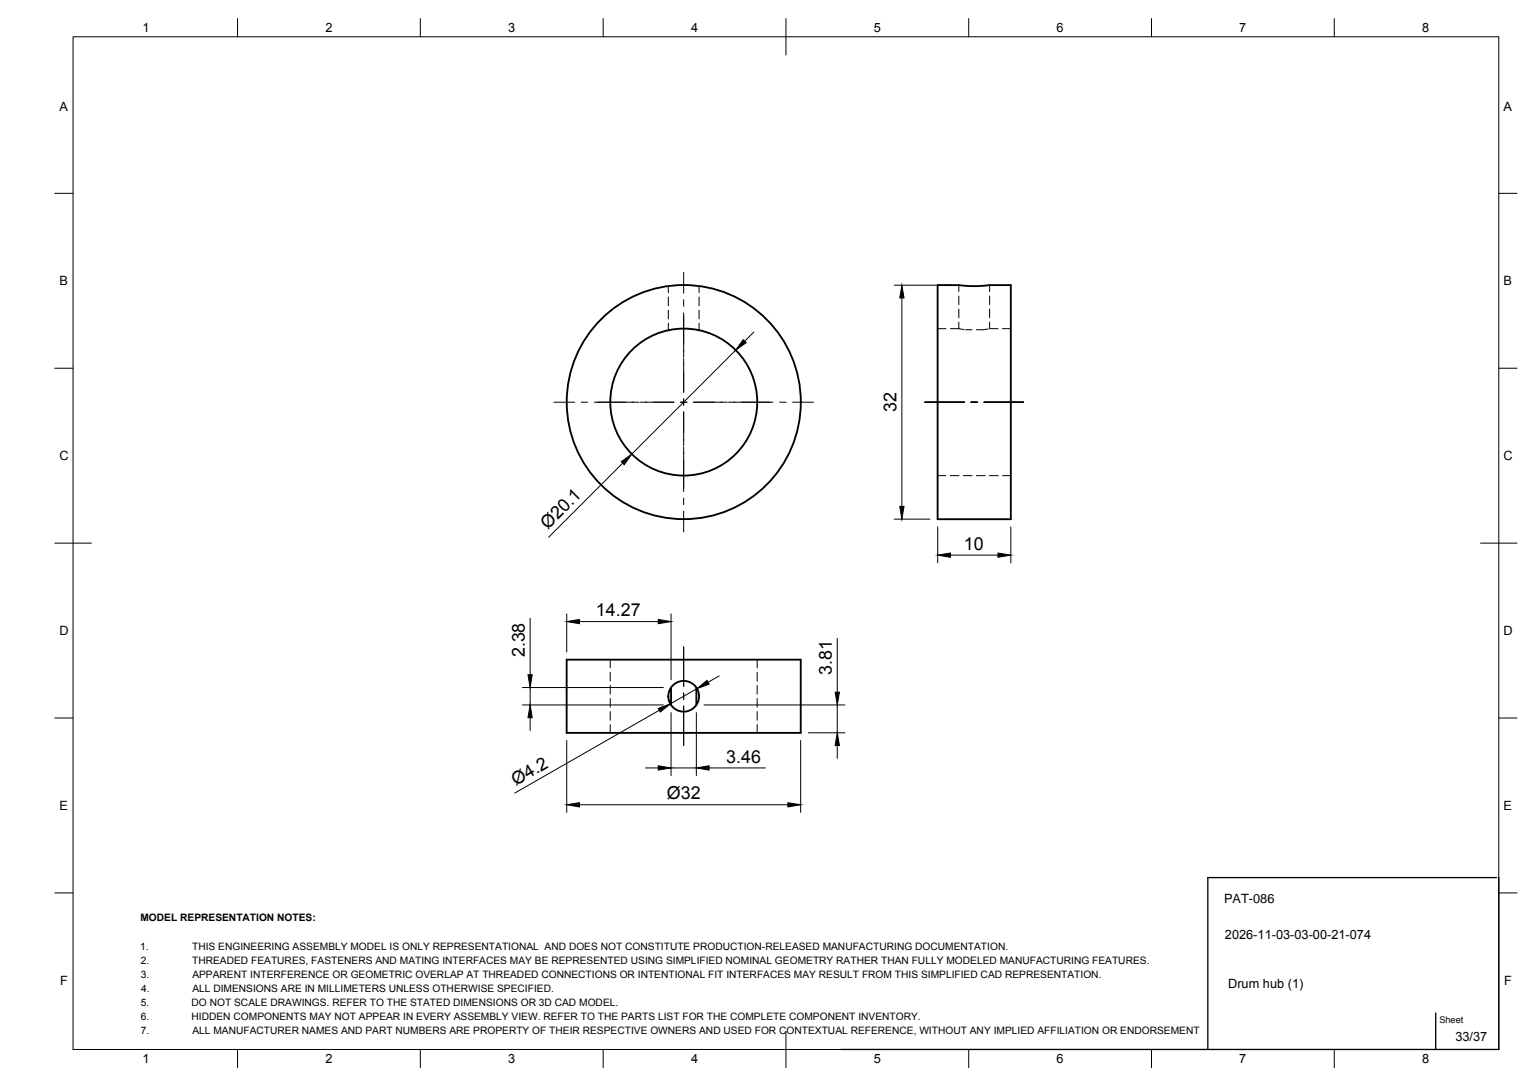
ISO-10303-21;
HEADER;
/* Generated by software containing ST-Developer
 * from STEP Tools, Inc. (www.steptools.com) 
 */

FILE_DESCRIPTION(
/* description */ ('Ratchet and pawl hand winch drum'),
/* implementation_level */ '2;1');

FILE_NAME(
/* name */ 'Drum hub (1).step',
/* time_stamp */ '2026-10-27T12:42:58-07:00',
/* author */ (''),
/* organization */ (''),
/* preprocessor_version */ 'ST-DEVELOPER v20.2',
/* originating_system */ 'Autodesk Translation Framework v15.17.0.0',
/* authorisation */ '');

FILE_SCHEMA (('AUTOMOTIVE_DESIGN { 1 0 10303 214 3 1 1 }'));
ENDSEC;

DATA;
#10=MECHANICAL_DESIGN_GEOMETRIC_PRESENTATION_REPRESENTATION('',(#417),#11801);
#309=B_SPLINE_CURVE_WITH_KNOTS('',3,(#10928,#10929,#10930,#10931,#10932,
#10933,#10934,#10935,#10936,#10937,#10938,#10939,#10940,#10941),
 .UNSPECIFIED.,.F.,.F.,(4,2,2,2,2,2,4),(0.756005737987023,0.793568827564648,
0.872922520054203,0.952276212543758,1.03162990503331,1.11098359752287,1.1485466871005),
 .UNSPECIFIED.);
#310=B_SPLINE_CURVE_WITH_KNOTS('',3,(#10947,#10948,#10949,#10950,#10951,
#10952,#10953,#10954,#10955,#10956,#10957,#10958,#10959,#10960,#10961,#10962,
#10963,#10964),.UNSPECIFIED.,.F.,.F.,(4,2,2,2,2,2,2,2,4),(0.,0.0792028026112442,
0.158405605222488,0.237607602356378,0.316809599490267,0.396011596624156,
0.475213593758046,0.55441639636929,0.633619198980534),.UNSPECIFIED.);
#311=B_SPLINE_CURVE_WITH_KNOTS('',3,(#10965,#10966,#10967,#10968,#10969,
#10970,#10971,#10972,#10973,#10974,#10975,#10976,#10977,#10978,#10979,#10980,
#10981,#10982),.UNSPECIFIED.,.F.,.F.,(4,2,2,2,2,2,2,2,4),(0.633619198980534,
0.712822001591778,0.792024804203022,0.871226801336912,0.950428798470801,
1.02963079560469,1.10883279273858,1.18803559534982,1.26723839796107),
 .UNSPECIFIED.);
#312=B_SPLINE_CURVE_WITH_KNOTS('',3,(#10985,#10986,#10987,#10988,#10989,
#10990,#10991,#10992,#10993,#10994,#10995,#10996,#10997,#10998),
 .UNSPECIFIED.,.F.,.F.,(4,2,2,2,2,2,4),(0.121154929624518,0.158718019202143,
0.238071711691698,0.317425404181253,0.396779096670807,0.476132789160362,
0.513695878737989),.UNSPECIFIED.);
#348=SHAPE_REPRESENTATION_RELATIONSHIP('SRR','None',#11976,#382);
#382=ADVANCED_BREP_SHAPE_REPRESENTATION('',(#450),#11793);
#417=STYLED_ITEM('',(#12199),#450);
#450=MANIFOLD_SOLID_BREP('Body1',#6296);
#582=FACE_BOUND('',#1565,.T.);
#583=FACE_BOUND('',#1567,.T.);
#584=FACE_BOUND('',#1569,.T.);
#585=FACE_BOUND('',#1571,.T.);
#746=PLANE('',#7129);
#747=PLANE('',#7134);
#748=PLANE('',#7141);
#749=PLANE('',#7142);
#1079=FACE_OUTER_BOUND('',#1561,.T.);
#1080=FACE_OUTER_BOUND('',#1562,.T.);
#1081=FACE_OUTER_BOUND('',#1563,.T.);
#1082=FACE_OUTER_BOUND('',#1564,.T.);
#1083=FACE_OUTER_BOUND('',#1566,.T.);
#1084=FACE_OUTER_BOUND('',#1568,.T.);
#1085=FACE_OUTER_BOUND('',#1570,.T.);
#1561=EDGE_LOOP('',(#5239,#5240));
#1562=EDGE_LOOP('',(#5241,#5242,#5243,#5244,#5245,#5246,#5247,#5248,#5249));
#1563=EDGE_LOOP('',(#5250,#5251,#5252));
#1564=EDGE_LOOP('',(#5253,#5254,#5255,#5256));
#1565=EDGE_LOOP('',(#5257,#5258,#5259,#5260));
#1566=EDGE_LOOP('',(#5261,#5262,#5263,#5264));
#1567=EDGE_LOOP('',(#5265,#5266));
#1568=EDGE_LOOP('',(#5267));
#1569=EDGE_LOOP('',(#5268));
#1570=EDGE_LOOP('',(#5269));
#1571=EDGE_LOOP('',(#5270));
#1980=LINE('',#10924,#2491);
#1981=LINE('',#10945,#2492);
#1982=LINE('',#11000,#2493);
#1983=LINE('',#11005,#2494);
#1984=LINE('',#11011,#2495);
#2491=VECTOR('',#8543,1.);
#2492=VECTOR('',#8550,0.21);
#2493=VECTOR('',#8555,1.);
#2494=VECTOR('',#8560,1.005);
#2495=VECTOR('',#8567,1.6);
#2896=CIRCLE('',#7130,0.21);
#2897=CIRCLE('',#7132,0.21);
#2898=CIRCLE('',#7133,0.21);
#2899=CIRCLE('',#7136,1.005);
#2900=CIRCLE('',#7137,1.005);
#2901=CIRCLE('',#7139,1.6);
#2902=CIRCLE('',#7140,1.6);
#3279=VERTEX_POINT('',#10922);
#3280=VERTEX_POINT('',#10923);
#3281=VERTEX_POINT('',#10927);
#3282=VERTEX_POINT('',#10942);
#3283=VERTEX_POINT('',#10944);
#3284=VERTEX_POINT('',#10946);
#3285=VERTEX_POINT('',#10983);
#3286=VERTEX_POINT('',#11002);
#3287=VERTEX_POINT('',#11004);
#3288=VERTEX_POINT('',#11008);
#3289=VERTEX_POINT('',#11010);
#3963=EDGE_CURVE('',#3279,#3280,#1980,.T.);
#3964=EDGE_CURVE('',#3279,#3280,#2896,.T.);
#3965=EDGE_CURVE('',#3281,#3279,#309,.T.);
#3966=EDGE_CURVE('',#3282,#3281,#2897,.T.);
#3967=EDGE_CURVE('',#3282,#3283,#1981,.T.);
#3968=EDGE_CURVE('',#3284,#3283,#310,.T.);
#3969=EDGE_CURVE('',#3283,#3284,#311,.T.);
#3970=EDGE_CURVE('',#3285,#3282,#2898,.T.);
#3971=EDGE_CURVE('',#3280,#3285,#312,.T.);
#3972=EDGE_CURVE('',#3285,#3281,#1982,.T.);
#3973=EDGE_CURVE('',#3286,#3286,#2899,.T.);
#3974=EDGE_CURVE('',#3286,#3287,#1983,.T.);
#3975=EDGE_CURVE('',#3287,#3287,#2900,.T.);
#3976=EDGE_CURVE('',#3288,#3288,#2901,.T.);
#3977=EDGE_CURVE('',#3288,#3289,#1984,.T.);
#3978=EDGE_CURVE('',#3289,#3289,#2902,.T.);
#5239=ORIENTED_EDGE('',*,*,#3963,.F.);
#5240=ORIENTED_EDGE('',*,*,#3964,.T.);
#5241=ORIENTED_EDGE('',*,*,#3965,.F.);
#5242=ORIENTED_EDGE('',*,*,#3966,.F.);
#5243=ORIENTED_EDGE('',*,*,#3967,.T.);
#5244=ORIENTED_EDGE('',*,*,#3968,.F.);
#5245=ORIENTED_EDGE('',*,*,#3969,.F.);
#5246=ORIENTED_EDGE('',*,*,#3967,.F.);
#5247=ORIENTED_EDGE('',*,*,#3970,.F.);
#5248=ORIENTED_EDGE('',*,*,#3971,.F.);
#5249=ORIENTED_EDGE('',*,*,#3964,.F.);
#5250=ORIENTED_EDGE('',*,*,#3972,.F.);
#5251=ORIENTED_EDGE('',*,*,#3970,.T.);
#5252=ORIENTED_EDGE('',*,*,#3966,.T.);
#5253=ORIENTED_EDGE('',*,*,#3973,.F.);
#5254=ORIENTED_EDGE('',*,*,#3974,.T.);
#5255=ORIENTED_EDGE('',*,*,#3975,.T.);
#5256=ORIENTED_EDGE('',*,*,#3974,.F.);
#5257=ORIENTED_EDGE('',*,*,#3971,.T.);
#5258=ORIENTED_EDGE('',*,*,#3972,.T.);
#5259=ORIENTED_EDGE('',*,*,#3965,.T.);
#5260=ORIENTED_EDGE('',*,*,#3963,.T.);
#5261=ORIENTED_EDGE('',*,*,#3976,.F.);
#5262=ORIENTED_EDGE('',*,*,#3977,.T.);
#5263=ORIENTED_EDGE('',*,*,#3978,.T.);
#5264=ORIENTED_EDGE('',*,*,#3977,.F.);
#5265=ORIENTED_EDGE('',*,*,#3968,.T.);
#5266=ORIENTED_EDGE('',*,*,#3969,.T.);
#5267=ORIENTED_EDGE('',*,*,#3976,.T.);
#5268=ORIENTED_EDGE('',*,*,#3973,.T.);
#5269=ORIENTED_EDGE('',*,*,#3978,.F.);
#5270=ORIENTED_EDGE('',*,*,#3975,.F.);
#5893=CYLINDRICAL_SURFACE('',#7131,0.21);
#5894=CYLINDRICAL_SURFACE('',#7135,1.005);
#5895=CYLINDRICAL_SURFACE('',#7138,1.6);
#6149=ADVANCED_FACE('',(#1079),#746,.T.);
#6150=ADVANCED_FACE('',(#1080),#5893,.F.);
#6151=ADVANCED_FACE('',(#1081),#747,.T.);
#6152=ADVANCED_FACE('',(#1082,#582),#5894,.F.);
#6153=ADVANCED_FACE('',(#1083,#583),#5895,.T.);
#6154=ADVANCED_FACE('',(#1084,#584),#748,.T.);
#6155=ADVANCED_FACE('',(#1085,#585),#749,.F.);
#6296=CLOSED_SHELL('',(#6149,#6150,#6151,#6152,#6153,#6154,#6155));
#7128=AXIS2_PLACEMENT_3D('',#10920,#8539,#8540);
#7129=AXIS2_PLACEMENT_3D('',#10921,#8541,#8542);
#7130=AXIS2_PLACEMENT_3D('',#10925,#8544,#8545);
#7131=AXIS2_PLACEMENT_3D('',#10926,#8546,#8547);
#7132=AXIS2_PLACEMENT_3D('',#10943,#8548,#8549);
#7133=AXIS2_PLACEMENT_3D('',#10984,#8551,#8552);
#7134=AXIS2_PLACEMENT_3D('',#10999,#8553,#8554);
#7135=AXIS2_PLACEMENT_3D('',#11001,#8556,#8557);
#7136=AXIS2_PLACEMENT_3D('',#11003,#8558,#8559);
#7137=AXIS2_PLACEMENT_3D('',#11006,#8561,#8562);
#7138=AXIS2_PLACEMENT_3D('',#11007,#8563,#8564);
#7139=AXIS2_PLACEMENT_3D('',#11009,#8565,#8566);
#7140=AXIS2_PLACEMENT_3D('',#11012,#8568,#8569);
#7141=AXIS2_PLACEMENT_3D('',#11013,#8570,#8571);
#7142=AXIS2_PLACEMENT_3D('',#11014,#8572,#8573);
#8539=DIRECTION('axis',(0.,0.,1.));
#8540=DIRECTION('refdir',(1.,0.,0.));
#8541=DIRECTION('center_axis',(0.,0.,1.));
#8542=DIRECTION('ref_axis',(1.,0.,0.));
#8543=DIRECTION('',(0.,1.,0.));
#8544=DIRECTION('center_axis',(0.,0.,1.));
#8545=DIRECTION('ref_axis',(1.,0.,0.));
#8546=DIRECTION('center_axis',(0.,0.,1.));
#8547=DIRECTION('ref_axis',(1.,0.,0.));
#8548=DIRECTION('center_axis',(0.,0.,1.));
#8549=DIRECTION('ref_axis',(1.,0.,0.));
#8550=DIRECTION('',(0.,0.,1.));
#8551=DIRECTION('center_axis',(0.,0.,1.));
#8552=DIRECTION('ref_axis',(1.,0.,0.));
#8553=DIRECTION('center_axis',(0.,0.,1.));
#8554=DIRECTION('ref_axis',(1.,0.,0.));
#8555=DIRECTION('',(0.,-1.,0.));
#8556=DIRECTION('center_axis',(0.,1.,0.));
#8557=DIRECTION('ref_axis',(1.,0.,0.));
#8558=DIRECTION('center_axis',(0.,-1.,0.));
#8559=DIRECTION('ref_axis',(1.,0.,0.));
#8560=DIRECTION('',(0.,-1.,0.));
#8561=DIRECTION('center_axis',(0.,-1.,0.));
#8562=DIRECTION('ref_axis',(1.,0.,0.));
#8563=DIRECTION('center_axis',(0.,1.,0.));
#8564=DIRECTION('ref_axis',(1.,0.,0.));
#8565=DIRECTION('center_axis',(0.,1.,0.));
#8566=DIRECTION('ref_axis',(1.,0.,0.));
#8567=DIRECTION('',(0.,-1.,0.));
#8568=DIRECTION('center_axis',(0.,1.,0.));
#8569=DIRECTION('ref_axis',(1.,0.,0.));
#8570=DIRECTION('center_axis',(0.,1.,0.));
#8571=DIRECTION('ref_axis',(1.,0.,0.));
#8572=DIRECTION('center_axis',(0.,1.,0.));
#8573=DIRECTION('ref_axis',(1.,0.,0.));
#10920=CARTESIAN_POINT('',(0.,0.,0.));
#10921=CARTESIAN_POINT('Origin',(0.,12.5,7.52));
#10922=CARTESIAN_POINT('',(0.172988438920056,12.3809411910021,7.52));
#10923=CARTESIAN_POINT('',(0.172988438920056,12.6190588089979,7.52));
#10924=CARTESIAN_POINT('',(0.172988438920056,12.,7.52));
#10925=CARTESIAN_POINT('Origin',(0.,12.5,7.52));
#10926=CARTESIAN_POINT('Origin',(0.,12.5,7.52));
#10927=CARTESIAN_POINT('',(-0.172988438920056,12.3809411910021,7.52));
#10928=CARTESIAN_POINT('Ctrl Pts',(-0.172988438920057,12.3809411910021,
7.52));
#10929=CARTESIAN_POINT('Ctrl Pts',(-0.165594865311316,12.3701985776047,
7.52129192197638));
#10930=CARTESIAN_POINT('Ctrl Pts',(-0.157297138725606,12.3603122906273,
7.52265394943905));
#10931=CARTESIAN_POINT('Ctrl Pts',(-0.129892073845076,12.3329072257467,
7.5267480843909));
#10932=CARTESIAN_POINT('Ctrl Pts',(-0.106330167759285,12.316757943667,7.52969589327638));
#10933=CARTESIAN_POINT('Ctrl Pts',(-0.0546129046324104,12.2953022060351,
7.53385029472357));
#10934=CARTESIAN_POINT('Ctrl Pts',(-0.0264512308298516,12.29,7.535));
#10935=CARTESIAN_POINT('Ctrl Pts',(0.0264512308298515,12.29,7.535));
#10936=CARTESIAN_POINT('Ctrl Pts',(0.0546129046324104,12.2953022060351,
7.53385029472357));
#10937=CARTESIAN_POINT('Ctrl Pts',(0.106330167759285,12.316757943667,7.52969589327638));
#10938=CARTESIAN_POINT('Ctrl Pts',(0.129892073845076,12.3329072257467,7.5267480843909));
#10939=CARTESIAN_POINT('Ctrl Pts',(0.157297138725607,12.3603122906273,7.52265394943905));
#10940=CARTESIAN_POINT('Ctrl Pts',(0.165594865311314,12.3701985776047,7.52129192197638));
#10941=CARTESIAN_POINT('Ctrl Pts',(0.172988438920056,12.3809411910021,7.52));
#10942=CARTESIAN_POINT('',(-0.21,12.5,7.52));
#10943=CARTESIAN_POINT('Origin',(0.,12.5,7.52));
#10944=CARTESIAN_POINT('',(-0.21,12.5,8.11615888233178));
#10945=CARTESIAN_POINT('',(-0.21,12.5,7.52));
#10946=CARTESIAN_POINT('',(0.21,12.5,8.11615888233178));
#10947=CARTESIAN_POINT('Ctrl Pts',(0.21,12.5,8.11615888233178));
#10948=CARTESIAN_POINT('Ctrl Pts',(0.21,12.4735990657963,8.11615888233178));
#10949=CARTESIAN_POINT('Ctrl Pts',(0.20471752266132,12.4454594446349,8.11688606295397));
#10950=CARTESIAN_POINT('Ctrl Pts',(0.183276841782292,12.3937289476995,8.11950502964782));
#10951=CARTESIAN_POINT('Ctrl Pts',(0.167120287247804,12.3701354391495,8.12135816887013));
#10952=CARTESIAN_POINT('Ctrl Pts',(0.129864750292352,12.332879902194,8.12483075953278));
#10953=CARTESIAN_POINT('Ctrl Pts',(0.106271159541075,12.3167231991688,8.12667690933009));
#10954=CARTESIAN_POINT('Ctrl Pts',(0.0545403836274679,12.2952824096556,
8.12927985626981));
#10955=CARTESIAN_POINT('Ctrl Pts',(0.0264006657112965,12.29,8.13));
#10956=CARTESIAN_POINT('Ctrl Pts',(-0.0264006657112964,12.29,8.13));
#10957=CARTESIAN_POINT('Ctrl Pts',(-0.0545403836274678,12.2952824096556,
8.12927985626981));
#10958=CARTESIAN_POINT('Ctrl Pts',(-0.106271159541075,12.3167231991688,
8.12667690933009));
#10959=CARTESIAN_POINT('Ctrl Pts',(-0.129864750292352,12.332879902194,8.12483075953278));
#10960=CARTESIAN_POINT('Ctrl Pts',(-0.167120287247804,12.3701354391495,
8.12135816887013));
#10961=CARTESIAN_POINT('Ctrl Pts',(-0.183276841782292,12.3937289476995,
8.11950502964782));
#10962=CARTESIAN_POINT('Ctrl Pts',(-0.20471752266132,12.4454594446349,8.11688606295397));
#10963=CARTESIAN_POINT('Ctrl Pts',(-0.21,12.4735990657963,8.11615888233178));
#10964=CARTESIAN_POINT('Ctrl Pts',(-0.21,12.5,8.11615888233178));
#10965=CARTESIAN_POINT('Ctrl Pts',(-0.21,12.5,8.11615888233178));
#10966=CARTESIAN_POINT('Ctrl Pts',(-0.21,12.5264009342037,8.11615888233178));
#10967=CARTESIAN_POINT('Ctrl Pts',(-0.20471752266132,12.5545405553651,8.11688606295397));
#10968=CARTESIAN_POINT('Ctrl Pts',(-0.183276841782292,12.6062710523005,
8.11950502964782));
#10969=CARTESIAN_POINT('Ctrl Pts',(-0.167120287247804,12.6298645608505,
8.12135816887013));
#10970=CARTESIAN_POINT('Ctrl Pts',(-0.129864750292352,12.667120097806,8.12483075953278));
#10971=CARTESIAN_POINT('Ctrl Pts',(-0.106271159541075,12.6832768008312,
8.12667690933009));
#10972=CARTESIAN_POINT('Ctrl Pts',(-0.0545403836274679,12.7047175903444,
8.12927985626981));
#10973=CARTESIAN_POINT('Ctrl Pts',(-0.0264006657112965,12.71,8.13));
#10974=CARTESIAN_POINT('Ctrl Pts',(0.0264006657112964,12.71,8.13));
#10975=CARTESIAN_POINT('Ctrl Pts',(0.0545403836274679,12.7047175903444,
8.12927985626981));
#10976=CARTESIAN_POINT('Ctrl Pts',(0.106271159541075,12.6832768008312,8.12667690933009));
#10977=CARTESIAN_POINT('Ctrl Pts',(0.129864750292352,12.667120097806,8.12483075953278));
#10978=CARTESIAN_POINT('Ctrl Pts',(0.167120287247804,12.6298645608505,8.12135816887013));
#10979=CARTESIAN_POINT('Ctrl Pts',(0.183276841782292,12.6062710523005,8.11950502964782));
#10980=CARTESIAN_POINT('Ctrl Pts',(0.20471752266132,12.5545405553651,8.11688606295397));
#10981=CARTESIAN_POINT('Ctrl Pts',(0.21,12.5264009342037,8.11615888233178));
#10982=CARTESIAN_POINT('Ctrl Pts',(0.21,12.5,8.11615888233178));
#10983=CARTESIAN_POINT('',(-0.172988438920056,12.6190588089979,7.52));
#10984=CARTESIAN_POINT('Origin',(0.,12.5,7.52));
#10985=CARTESIAN_POINT('Ctrl Pts',(0.172988438920056,12.6190588089979,7.52));
#10986=CARTESIAN_POINT('Ctrl Pts',(0.165594865311315,12.6298014223953,7.52129192197638));
#10987=CARTESIAN_POINT('Ctrl Pts',(0.157297138725606,12.6396877093727,7.52265394943905));
#10988=CARTESIAN_POINT('Ctrl Pts',(0.129892073845076,12.6670927742533,7.5267480843909));
#10989=CARTESIAN_POINT('Ctrl Pts',(0.106330167759285,12.683242056333,7.52969589327638));
#10990=CARTESIAN_POINT('Ctrl Pts',(0.0546129046324104,12.7046977939649,
7.53385029472357));
#10991=CARTESIAN_POINT('Ctrl Pts',(0.0264512308298516,12.71,7.535));
#10992=CARTESIAN_POINT('Ctrl Pts',(-0.0264512308298516,12.71,7.535));
#10993=CARTESIAN_POINT('Ctrl Pts',(-0.0546129046324104,12.7046977939649,
7.53385029472357));
#10994=CARTESIAN_POINT('Ctrl Pts',(-0.106330167759285,12.683242056333,7.52969589327638));
#10995=CARTESIAN_POINT('Ctrl Pts',(-0.129892073845076,12.6670927742533,
7.5267480843909));
#10996=CARTESIAN_POINT('Ctrl Pts',(-0.157297138725606,12.6396877093727,
7.52265394943905));
#10997=CARTESIAN_POINT('Ctrl Pts',(-0.165594865311316,12.6298014223953,
7.52129192197638));
#10998=CARTESIAN_POINT('Ctrl Pts',(-0.172988438920056,12.6190588089979,
7.52));
#10999=CARTESIAN_POINT('Origin',(0.,12.5,7.52));
#11000=CARTESIAN_POINT('',(-0.172988438920056,12.,7.52));
#11001=CARTESIAN_POINT('Origin',(0.,12.,6.53));
#11002=CARTESIAN_POINT('',(-1.005,13.,6.53));
#11003=CARTESIAN_POINT('Origin',(0.,13.,6.53));
#11004=CARTESIAN_POINT('',(-1.005,12.,6.53));
#11005=CARTESIAN_POINT('',(-1.005,12.,6.53));
#11006=CARTESIAN_POINT('Origin',(0.,12.,6.53));
#11007=CARTESIAN_POINT('Origin',(0.,12.,6.53));
#11008=CARTESIAN_POINT('',(-1.6,13.,6.53));
#11009=CARTESIAN_POINT('Origin',(0.,13.,6.53));
#11010=CARTESIAN_POINT('',(-1.6,12.,6.53));
#11011=CARTESIAN_POINT('',(-1.6,12.,6.53));
#11012=CARTESIAN_POINT('Origin',(0.,12.,6.53));
#11013=CARTESIAN_POINT('Origin',(0.,13.,6.53));
#11014=CARTESIAN_POINT('Origin',(0.,12.,6.53));
#11753=UNCERTAINTY_MEASURE_WITH_UNIT(LENGTH_MEASURE(0.001),#11802,
'DISTANCE_ACCURACY_VALUE',
'Maximum model space distance between geometric entities at asserted c
onnectivities');
#11761=UNCERTAINTY_MEASURE_WITH_UNIT(LENGTH_MEASURE(0.001),#11802,
'DISTANCE_ACCURACY_VALUE',
'Maximum model space distance between geometric entities at asserted c
onnectivities');
#11793=(
GEOMETRIC_REPRESENTATION_CONTEXT(3)
GLOBAL_UNCERTAINTY_ASSIGNED_CONTEXT((#11753))
GLOBAL_UNIT_ASSIGNED_CONTEXT((#11802,#11804,#11805))
REPRESENTATION_CONTEXT('','3D')
);
#11801=(
GEOMETRIC_REPRESENTATION_CONTEXT(3)
GLOBAL_UNCERTAINTY_ASSIGNED_CONTEXT((#11761))
GLOBAL_UNIT_ASSIGNED_CONTEXT((#11802,#11804,#11805))
REPRESENTATION_CONTEXT('','3D')
);
#11802=(
LENGTH_UNIT()
NAMED_UNIT(*)
SI_UNIT(.CENTI.,.METRE.)
);
#11804=(
NAMED_UNIT(*)
PLANE_ANGLE_UNIT()
SI_UNIT($,.RADIAN.)
);
#11805=(
NAMED_UNIT(*)
SI_UNIT($,.STERADIAN.)
SOLID_ANGLE_UNIT()
);
#11837=SHAPE_DEFINITION_REPRESENTATION(#11878,#11976);
#11878=PRODUCT_DEFINITION_SHAPE('',$,#12016);
#11976=SHAPE_REPRESENTATION('',(#7128),#11793);
#11984=PRODUCT_DEFINITION_CONTEXT('part definition',#12103,'design');
#12016=PRODUCT_DEFINITION('Drum hub (1)','Drum hub (1)',#12055,#11984);
#12055=PRODUCT_DEFINITION_FORMATION('',$,#12136);
#12103=APPLICATION_CONTEXT(
'Core Data for Automotive Mechanical Design Process');
#12104=PRODUCT_CONTEXT('part definition',#12103,'mechanical');
#12136=PRODUCT('Drum hub (1)','Drum hub (1)','Drum hub (1)',(#12104));
#12193=COLOUR_RGB('Light Blue',0.38,0.62,0.78);
#12194=FILL_AREA_STYLE_COLOUR('',#12193);
#12195=FILL_AREA_STYLE('',(#12194));
#12196=SURFACE_STYLE_FILL_AREA(#12195);
#12197=SURFACE_SIDE_STYLE('',(#12196));
#12198=SURFACE_STYLE_USAGE(.BOTH.,#12197);
#12199=PRESENTATION_STYLE_ASSIGNMENT((#12198));
ENDSEC;
END-ISO-10303-21;
